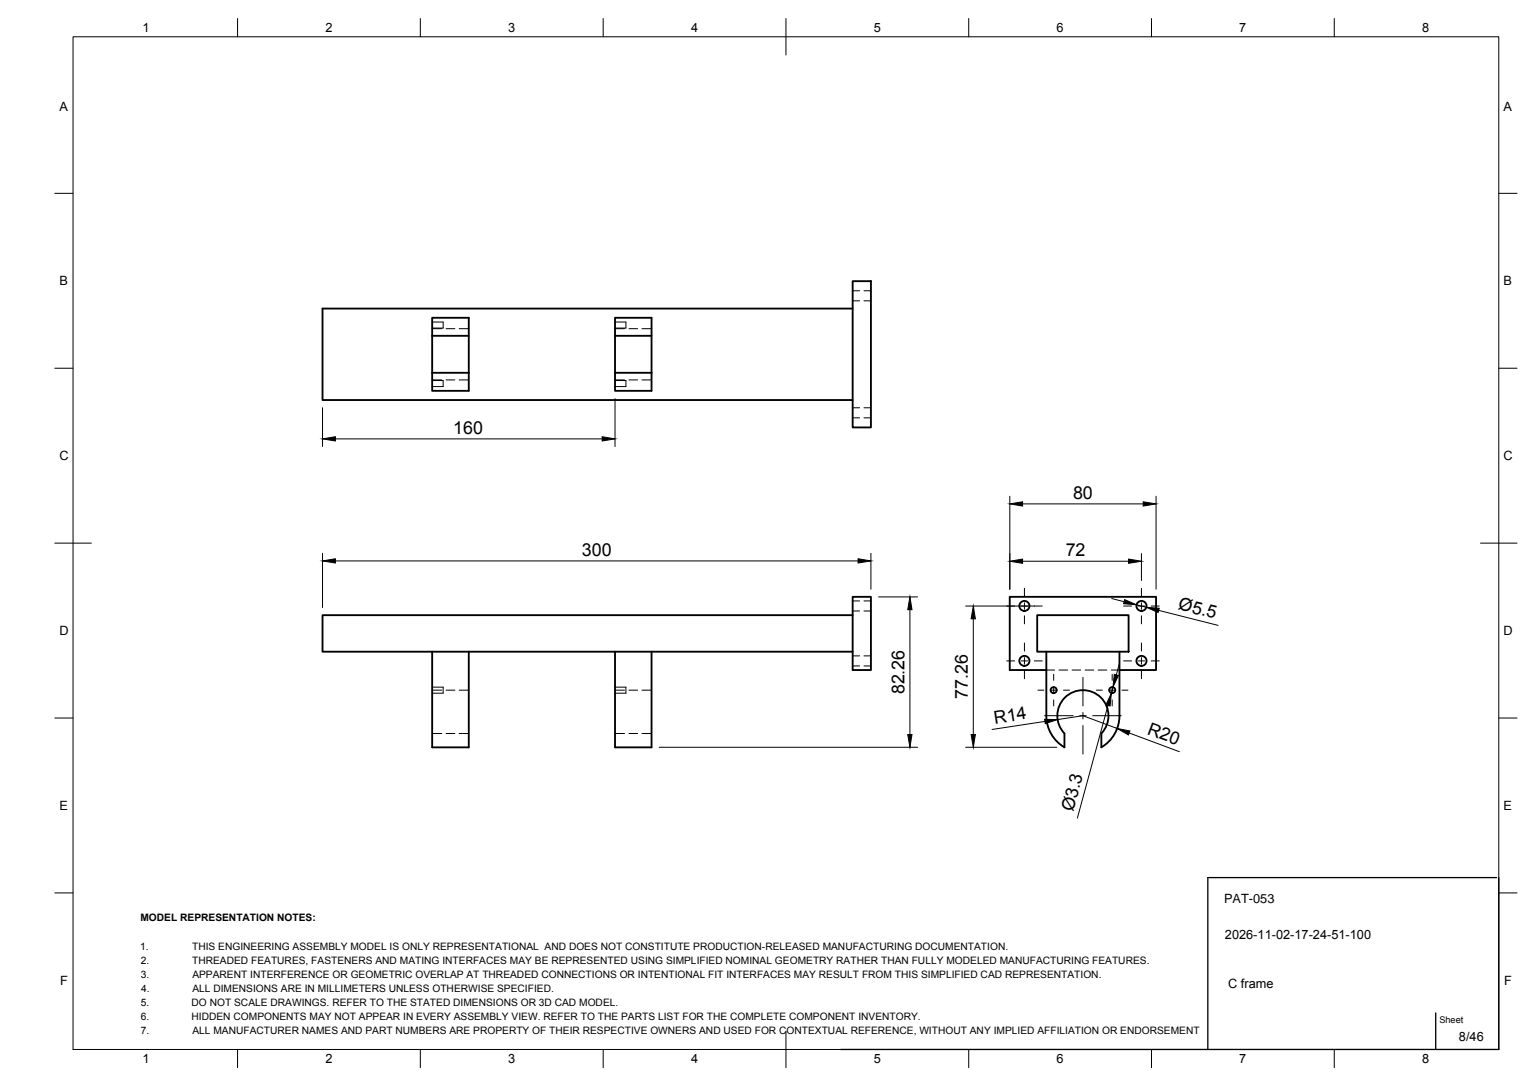
ISO-10303-21;
HEADER;
/* Generated by software containing ST-Developer
 * from STEP Tools, Inc. (www.steptools.com) 
 */

FILE_DESCRIPTION(
/* description */ ('Hand-operated arbor press'),
/* implementation_level */ '2;1');

FILE_NAME(
/* name */ 'C frame.step',
/* time_stamp */ '2026-10-28T03:25:25-07:00',
/* author */ (''),
/* organization */ (''),
/* preprocessor_version */ 'ST-DEVELOPER v20.2',
/* originating_system */ 'Autodesk Translation Framework v15.17.0.0',
/* authorisation */ '');

FILE_SCHEMA (('AUTOMOTIVE_DESIGN { 1 0 10303 214 3 1 1 }'));
ENDSEC;

DATA;
#10=MECHANICAL_DESIGN_GEOMETRIC_PRESENTATION_REPRESENTATION('',(#589),#32751);
#505=SHAPE_REPRESENTATION_RELATIONSHIP('SRR','None',#32934,#547);
#547=ADVANCED_BREP_SHAPE_REPRESENTATION('',(#638),#32708);
#589=STYLED_ITEM('',(#33221),#638);
#638=MANIFOLD_SOLID_BREP('Body1',#12486);
#700=FACE_BOUND('',#2033,.T.);
#701=FACE_BOUND('',#2034,.T.);
#702=FACE_BOUND('',#2048,.T.);
#703=FACE_BOUND('',#2049,.T.);
#704=FACE_BOUND('',#2057,.T.);
#705=FACE_BOUND('',#2058,.T.);
#706=FACE_BOUND('',#2059,.T.);
#707=FACE_BOUND('',#2060,.T.);
#708=FACE_BOUND('',#2061,.T.);
#709=FACE_BOUND('',#2070,.T.);
#710=FACE_BOUND('',#2071,.T.);
#711=FACE_BOUND('',#2074,.T.);
#712=FACE_BOUND('',#2075,.T.);
#713=FACE_BOUND('',#2076,.T.);
#714=FACE_BOUND('',#2077,.T.);
#867=PLANE('',#13056);
#868=PLANE('',#13060);
#869=PLANE('',#13061);
#870=PLANE('',#13062);
#871=PLANE('',#13063);
#872=PLANE('',#13073);
#873=PLANE('',#13074);
#874=PLANE('',#13075);
#875=PLANE('',#13079);
#876=PLANE('',#13083);
#877=PLANE('',#13084);
#878=PLANE('',#13085);
#879=PLANE('',#13086);
#880=PLANE('',#13096);
#881=PLANE('',#13097);
#882=PLANE('',#13098);
#883=PLANE('',#13111);
#884=PLANE('',#13112);
#885=PLANE('',#13113);
#886=PLANE('',#13114);
#887=PLANE('',#13115);
#888=PLANE('',#13116);
#889=PLANE('',#13117);
#890=PLANE('',#13118);
#891=PLANE('',#13119);
#892=PLANE('',#13120);
#893=PLANE('',#13121);
#1321=FACE_OUTER_BOUND('',#2022,.T.);
#1322=FACE_OUTER_BOUND('',#2023,.T.);
#1323=FACE_OUTER_BOUND('',#2024,.T.);
#1324=FACE_OUTER_BOUND('',#2025,.T.);
#1325=FACE_OUTER_BOUND('',#2026,.T.);
#1326=FACE_OUTER_BOUND('',#2027,.T.);
#1327=FACE_OUTER_BOUND('',#2028,.T.);
#1328=FACE_OUTER_BOUND('',#2029,.T.);
#1329=FACE_OUTER_BOUND('',#2030,.T.);
#1330=FACE_OUTER_BOUND('',#2031,.T.);
#1331=FACE_OUTER_BOUND('',#2032,.T.);
#1332=FACE_OUTER_BOUND('',#2035,.T.);
#1333=FACE_OUTER_BOUND('',#2036,.T.);
#1334=FACE_OUTER_BOUND('',#2037,.T.);
#1335=FACE_OUTER_BOUND('',#2038,.T.);
#1336=FACE_OUTER_BOUND('',#2039,.T.);
#1337=FACE_OUTER_BOUND('',#2040,.T.);
#1338=FACE_OUTER_BOUND('',#2041,.T.);
#1339=FACE_OUTER_BOUND('',#2042,.T.);
#1340=FACE_OUTER_BOUND('',#2043,.T.);
#1341=FACE_OUTER_BOUND('',#2044,.T.);
#1342=FACE_OUTER_BOUND('',#2045,.T.);
#1343=FACE_OUTER_BOUND('',#2046,.T.);
#1344=FACE_OUTER_BOUND('',#2047,.T.);
#1345=FACE_OUTER_BOUND('',#2050,.T.);
#1346=FACE_OUTER_BOUND('',#2051,.T.);
#1347=FACE_OUTER_BOUND('',#2052,.T.);
#1348=FACE_OUTER_BOUND('',#2053,.T.);
#1349=FACE_OUTER_BOUND('',#2054,.T.);
#1350=FACE_OUTER_BOUND('',#2055,.T.);
#1351=FACE_OUTER_BOUND('',#2056,.T.);
#1352=FACE_OUTER_BOUND('',#2062,.T.);
#1353=FACE_OUTER_BOUND('',#2063,.T.);
#1354=FACE_OUTER_BOUND('',#2064,.T.);
#1355=FACE_OUTER_BOUND('',#2065,.T.);
#1356=FACE_OUTER_BOUND('',#2066,.T.);
#1357=FACE_OUTER_BOUND('',#2067,.T.);
#1358=FACE_OUTER_BOUND('',#2068,.T.);
#1359=FACE_OUTER_BOUND('',#2069,.T.);
#1360=FACE_OUTER_BOUND('',#2072,.T.);
#1361=FACE_OUTER_BOUND('',#2073,.T.);
#2022=EDGE_LOOP('',(#8456,#8457,#8458,#8459));
#2023=EDGE_LOOP('',(#8460));
#2024=EDGE_LOOP('',(#8461,#8462,#8463,#8464));
#2025=EDGE_LOOP('',(#8465));
#2026=EDGE_LOOP('',(#8466,#8467,#8468,#8469));
#2027=EDGE_LOOP('',(#8470,#8471,#8472,#8473));
#2028=EDGE_LOOP('',(#8474,#8475,#8476,#8477,#8478,#8479,#8480,#8481));
#2029=EDGE_LOOP('',(#8482,#8483,#8484,#8485));
#2030=EDGE_LOOP('',(#8486,#8487,#8488,#8489));
#2031=EDGE_LOOP('',(#8490,#8491,#8492,#8493));
#2032=EDGE_LOOP('',(#8494,#8495,#8496,#8497,#8498,#8499,#8500,#8501));
#2033=EDGE_LOOP('',(#8502));
#2034=EDGE_LOOP('',(#8503));
#2035=EDGE_LOOP('',(#8504,#8505,#8506,#8507));
#2036=EDGE_LOOP('',(#8508,#8509,#8510,#8511));
#2037=EDGE_LOOP('',(#8512,#8513,#8514,#8515));
#2038=EDGE_LOOP('',(#8516));
#2039=EDGE_LOOP('',(#8517,#8518,#8519,#8520));
#2040=EDGE_LOOP('',(#8521));
#2041=EDGE_LOOP('',(#8522,#8523,#8524,#8525));
#2042=EDGE_LOOP('',(#8526,#8527,#8528,#8529));
#2043=EDGE_LOOP('',(#8530,#8531,#8532,#8533,#8534,#8535,#8536,#8537));
#2044=EDGE_LOOP('',(#8538,#8539,#8540,#8541));
#2045=EDGE_LOOP('',(#8542,#8543,#8544,#8545));
#2046=EDGE_LOOP('',(#8546,#8547,#8548,#8549));
#2047=EDGE_LOOP('',(#8550,#8551,#8552,#8553,#8554,#8555,#8556,#8557));
#2048=EDGE_LOOP('',(#8558));
#2049=EDGE_LOOP('',(#8559));
#2050=EDGE_LOOP('',(#8560,#8561,#8562,#8563));
#2051=EDGE_LOOP('',(#8564,#8565,#8566,#8567));
#2052=EDGE_LOOP('',(#8568,#8569,#8570,#8571));
#2053=EDGE_LOOP('',(#8572,#8573,#8574,#8575));
#2054=EDGE_LOOP('',(#8576,#8577,#8578,#8579));
#2055=EDGE_LOOP('',(#8580,#8581,#8582,#8583));
#2056=EDGE_LOOP('',(#8584,#8585,#8586,#8587));
#2057=EDGE_LOOP('',(#8588,#8589,#8590,#8591));
#2058=EDGE_LOOP('',(#8592));
#2059=EDGE_LOOP('',(#8593));
#2060=EDGE_LOOP('',(#8594));
#2061=EDGE_LOOP('',(#8595));
#2062=EDGE_LOOP('',(#8596,#8597,#8598,#8599));
#2063=EDGE_LOOP('',(#8600,#8601,#8602,#8603));
#2064=EDGE_LOOP('',(#8604,#8605,#8606,#8607));
#2065=EDGE_LOOP('',(#8608,#8609,#8610,#8611));
#2066=EDGE_LOOP('',(#8612,#8613,#8614,#8615));
#2067=EDGE_LOOP('',(#8616,#8617,#8618,#8619));
#2068=EDGE_LOOP('',(#8620,#8621,#8622,#8623));
#2069=EDGE_LOOP('',(#8624,#8625,#8626,#8627));
#2070=EDGE_LOOP('',(#8628,#8629,#8630,#8631));
#2071=EDGE_LOOP('',(#8632,#8633,#8634,#8635));
#2072=EDGE_LOOP('',(#8636,#8637,#8638,#8639));
#2073=EDGE_LOOP('',(#8640,#8641,#8642,#8643));
#2074=EDGE_LOOP('',(#8644));
#2075=EDGE_LOOP('',(#8645));
#2076=EDGE_LOOP('',(#8646));
#2077=EDGE_LOOP('',(#8647));
#2870=LINE('',#17786,#4041);
#2871=LINE('',#17793,#4042);
#2872=LINE('',#17799,#4043);
#2873=LINE('',#17801,#4044);
#2874=LINE('',#17803,#4045);
#2875=LINE('',#17804,#4046);
#2876=LINE('',#17808,#4047);
#2877=LINE('',#17810,#4048);
#2878=LINE('',#17812,#4049);
#2879=LINE('',#17813,#4050);
#2880=LINE('',#17818,#4051);
#2881=LINE('',#17820,#4052);
#2882=LINE('',#17822,#4053);
#2883=LINE('',#17829,#4054);
#2884=LINE('',#17834,#4055);
#2885=LINE('',#17837,#4056);
#2886=LINE('',#17839,#4057);
#2887=LINE('',#17840,#4058);
#2888=LINE('',#17842,#4059);
#2889=LINE('',#17844,#4060);
#2890=LINE('',#17849,#4061);
#2891=LINE('',#17856,#4062);
#2892=LINE('',#17862,#4063);
#2893=LINE('',#17864,#4064);
#2894=LINE('',#17866,#4065);
#2895=LINE('',#17867,#4066);
#2896=LINE('',#17871,#4067);
#2897=LINE('',#17873,#4068);
#2898=LINE('',#17875,#4069);
#2899=LINE('',#17876,#4070);
#2900=LINE('',#17881,#4071);
#2901=LINE('',#17883,#4072);
#2902=LINE('',#17885,#4073);
#2903=LINE('',#17892,#4074);
#2904=LINE('',#17897,#4075);
#2905=LINE('',#17900,#4076);
#2906=LINE('',#17902,#4077);
#2907=LINE('',#17903,#4078);
#2908=LINE('',#17905,#4079);
#2909=LINE('',#17907,#4080);
#2910=LINE('',#17912,#4081);
#2911=LINE('',#17918,#4082);
#2912=LINE('',#17924,#4083);
#2913=LINE('',#17930,#4084);
#2914=LINE('',#17935,#4085);
#2915=LINE('',#17937,#4086);
#2916=LINE('',#17939,#4087);
#2917=LINE('',#17940,#4088);
#2918=LINE('',#17943,#4089);
#2919=LINE('',#17945,#4090);
#2920=LINE('',#17947,#4091);
#2921=LINE('',#17948,#4092);
#2922=LINE('',#17952,#4093);
#2923=LINE('',#17953,#4094);
#2924=LINE('',#17954,#4095);
#2925=LINE('',#17957,#4096);
#2926=LINE('',#17958,#4097);
#2927=LINE('',#17961,#4098);
#2928=LINE('',#17962,#4099);
#2929=LINE('',#17964,#4100);
#2930=LINE('',#17967,#4101);
#2931=LINE('',#17969,#4102);
#2932=LINE('',#17970,#4103);
#2933=LINE('',#17973,#4104);
#2934=LINE('',#17974,#4105);
#2935=LINE('',#17977,#4106);
#2936=LINE('',#17978,#4107);
#2937=LINE('',#17980,#4108);
#4041=VECTOR('',#14313,0.165);
#4042=VECTOR('',#14322,0.165);
#4043=VECTOR('',#14329,1.);
#4044=VECTOR('',#14330,1.);
#4045=VECTOR('',#14331,1.);
#4046=VECTOR('',#14332,1.);
#4047=VECTOR('',#14335,1.);
#4048=VECTOR('',#14336,1.);
#4049=VECTOR('',#14337,1.);
#4050=VECTOR('',#14338,1.);
#4051=VECTOR('',#14343,1.);
#4052=VECTOR('',#14344,1.);
#4053=VECTOR('',#14345,1.);
#4054=VECTOR('',#14356,1.);
#4055=VECTOR('',#14363,1.);
#4056=VECTOR('',#14366,1.);
#4057=VECTOR('',#14367,1.);
#4058=VECTOR('',#14368,1.);
#4059=VECTOR('',#14371,1.);
#4060=VECTOR('',#14374,1.);
#4061=VECTOR('',#14379,0.165);
#4062=VECTOR('',#14388,0.165);
#4063=VECTOR('',#14395,1.);
#4064=VECTOR('',#14396,1.);
#4065=VECTOR('',#14397,1.);
#4066=VECTOR('',#14398,1.);
#4067=VECTOR('',#14401,1.);
#4068=VECTOR('',#14402,1.);
#4069=VECTOR('',#14403,1.);
#4070=VECTOR('',#14404,1.);
#4071=VECTOR('',#14409,1.);
#4072=VECTOR('',#14410,1.);
#4073=VECTOR('',#14411,1.);
#4074=VECTOR('',#14422,1.);
#4075=VECTOR('',#14429,1.);
#4076=VECTOR('',#14432,1.);
#4077=VECTOR('',#14433,1.);
#4078=VECTOR('',#14434,1.);
#4079=VECTOR('',#14437,1.);
#4080=VECTOR('',#14440,1.);
#4081=VECTOR('',#14445,0.275);
#4082=VECTOR('',#14452,0.275);
#4083=VECTOR('',#14459,0.275);
#4084=VECTOR('',#14466,0.275);
#4085=VECTOR('',#14471,1.);
#4086=VECTOR('',#14472,1.);
#4087=VECTOR('',#14473,1.);
#4088=VECTOR('',#14474,1.);
#4089=VECTOR('',#14475,1.);
#4090=VECTOR('',#14476,1.);
#4091=VECTOR('',#14477,1.);
#4092=VECTOR('',#14478,1.);
#4093=VECTOR('',#14481,1.);
#4094=VECTOR('',#14482,1.);
#4095=VECTOR('',#14483,1.);
#4096=VECTOR('',#14486,1.);
#4097=VECTOR('',#14487,1.);
#4098=VECTOR('',#14490,1.);
#4099=VECTOR('',#14491,1.);
#4100=VECTOR('',#14494,1.);
#4101=VECTOR('',#14497,1.);
#4102=VECTOR('',#14498,1.);
#4103=VECTOR('',#14499,1.);
#4104=VECTOR('',#14502,1.);
#4105=VECTOR('',#14503,1.);
#4106=VECTOR('',#14506,1.);
#4107=VECTOR('',#14507,1.);
#4108=VECTOR('',#14510,1.);
#5186=CIRCLE('',#13054,0.165);
#5187=CIRCLE('',#13055,0.165);
#5188=CIRCLE('',#13058,0.165);
#5189=CIRCLE('',#13059,0.165);
#5190=CIRCLE('',#13064,2.);
#5191=CIRCLE('',#13065,2.);
#5192=CIRCLE('',#13066,1.4);
#5193=CIRCLE('',#13068,1.4);
#5194=CIRCLE('',#13070,2.);
#5195=CIRCLE('',#13072,2.);
#5196=CIRCLE('',#13077,0.165);
#5197=CIRCLE('',#13078,0.165);
#5198=CIRCLE('',#13081,0.165);
#5199=CIRCLE('',#13082,0.165);
#5200=CIRCLE('',#13087,2.);
#5201=CIRCLE('',#13088,2.);
#5202=CIRCLE('',#13089,1.4);
#5203=CIRCLE('',#13091,1.4);
#5204=CIRCLE('',#13093,2.);
#5205=CIRCLE('',#13095,2.);
#5206=CIRCLE('',#13100,0.275);
#5207=CIRCLE('',#13101,0.275);
#5208=CIRCLE('',#13103,0.275);
#5209=CIRCLE('',#13104,0.275);
#5210=CIRCLE('',#13106,0.275);
#5211=CIRCLE('',#13107,0.275);
#5212=CIRCLE('',#13109,0.275);
#5213=CIRCLE('',#13110,0.275);
#5600=VERTEX_POINT('',#17783);
#5601=VERTEX_POINT('',#17785);
#5602=VERTEX_POINT('',#17790);
#5603=VERTEX_POINT('',#17792);
#5604=VERTEX_POINT('',#17797);
#5605=VERTEX_POINT('',#17798);
#5606=VERTEX_POINT('',#17800);
#5607=VERTEX_POINT('',#17802);
#5608=VERTEX_POINT('',#17806);
#5609=VERTEX_POINT('',#17807);
#5610=VERTEX_POINT('',#17809);
#5611=VERTEX_POINT('',#17811);
#5612=VERTEX_POINT('',#17815);
#5613=VERTEX_POINT('',#17817);
#5614=VERTEX_POINT('',#17819);
#5615=VERTEX_POINT('',#17821);
#5616=VERTEX_POINT('',#17828);
#5617=VERTEX_POINT('',#17832);
#5618=VERTEX_POINT('',#17836);
#5619=VERTEX_POINT('',#17838);
#5620=VERTEX_POINT('',#17846);
#5621=VERTEX_POINT('',#17848);
#5622=VERTEX_POINT('',#17853);
#5623=VERTEX_POINT('',#17855);
#5624=VERTEX_POINT('',#17860);
#5625=VERTEX_POINT('',#17861);
#5626=VERTEX_POINT('',#17863);
#5627=VERTEX_POINT('',#17865);
#5628=VERTEX_POINT('',#17869);
#5629=VERTEX_POINT('',#17870);
#5630=VERTEX_POINT('',#17872);
#5631=VERTEX_POINT('',#17874);
#5632=VERTEX_POINT('',#17878);
#5633=VERTEX_POINT('',#17880);
#5634=VERTEX_POINT('',#17882);
#5635=VERTEX_POINT('',#17884);
#5636=VERTEX_POINT('',#17891);
#5637=VERTEX_POINT('',#17895);
#5638=VERTEX_POINT('',#17899);
#5639=VERTEX_POINT('',#17901);
#5640=VERTEX_POINT('',#17909);
#5641=VERTEX_POINT('',#17911);
#5642=VERTEX_POINT('',#17915);
#5643=VERTEX_POINT('',#17917);
#5644=VERTEX_POINT('',#17921);
#5645=VERTEX_POINT('',#17923);
#5646=VERTEX_POINT('',#17927);
#5647=VERTEX_POINT('',#17929);
#5648=VERTEX_POINT('',#17933);
#5649=VERTEX_POINT('',#17934);
#5650=VERTEX_POINT('',#17936);
#5651=VERTEX_POINT('',#17938);
#5652=VERTEX_POINT('',#17941);
#5653=VERTEX_POINT('',#17942);
#5654=VERTEX_POINT('',#17944);
#5655=VERTEX_POINT('',#17946);
#5656=VERTEX_POINT('',#17950);
#5657=VERTEX_POINT('',#17951);
#5658=VERTEX_POINT('',#17956);
#5659=VERTEX_POINT('',#17960);
#5660=VERTEX_POINT('',#17966);
#5661=VERTEX_POINT('',#17968);
#5662=VERTEX_POINT('',#17972);
#5663=VERTEX_POINT('',#17976);
#6731=EDGE_CURVE('',#5600,#5600,#5186,.T.);
#6732=EDGE_CURVE('',#5600,#5601,#2870,.T.);
#6733=EDGE_CURVE('',#5601,#5601,#5187,.T.);
#6734=EDGE_CURVE('',#5602,#5602,#5188,.T.);
#6735=EDGE_CURVE('',#5602,#5603,#2871,.T.);
#6736=EDGE_CURVE('',#5603,#5603,#5189,.T.);
#6737=EDGE_CURVE('',#5604,#5605,#2872,.T.);
#6738=EDGE_CURVE('',#5606,#5604,#2873,.T.);
#6739=EDGE_CURVE('',#5607,#5606,#2874,.T.);
#6740=EDGE_CURVE('',#5605,#5607,#2875,.T.);
#6741=EDGE_CURVE('',#5608,#5609,#2876,.T.);
#6742=EDGE_CURVE('',#5610,#5608,#2877,.T.);
#6743=EDGE_CURVE('',#5611,#5610,#2878,.T.);
#6744=EDGE_CURVE('',#5609,#5611,#2879,.T.);
#6745=EDGE_CURVE('',#5612,#5604,#5190,.T.);
#6746=EDGE_CURVE('',#5613,#5612,#2880,.T.);
#6747=EDGE_CURVE('',#5614,#5613,#2881,.T.);
#6748=EDGE_CURVE('',#5615,#5614,#2882,.T.);
#6749=EDGE_CURVE('',#5609,#5615,#5191,.T.);
#6750=EDGE_CURVE('',#5611,#5606,#5192,.T.);
#6751=EDGE_CURVE('',#5607,#5610,#5193,.T.);
#6752=EDGE_CURVE('',#5615,#5616,#2883,.T.);
#6753=EDGE_CURVE('',#5608,#5616,#5194,.T.);
#6754=EDGE_CURVE('',#5617,#5605,#5195,.T.);
#6755=EDGE_CURVE('',#5612,#5617,#2884,.T.);
#6756=EDGE_CURVE('',#5616,#5618,#2885,.T.);
#6757=EDGE_CURVE('',#5619,#5618,#2886,.T.);
#6758=EDGE_CURVE('',#5619,#5617,#2887,.T.);
#6759=EDGE_CURVE('',#5618,#5614,#2888,.T.);
#6760=EDGE_CURVE('',#5613,#5619,#2889,.T.);
#6761=EDGE_CURVE('',#5620,#5620,#5196,.T.);
#6762=EDGE_CURVE('',#5620,#5621,#2890,.T.);
#6763=EDGE_CURVE('',#5621,#5621,#5197,.T.);
#6764=EDGE_CURVE('',#5622,#5622,#5198,.T.);
#6765=EDGE_CURVE('',#5622,#5623,#2891,.T.);
#6766=EDGE_CURVE('',#5623,#5623,#5199,.T.);
#6767=EDGE_CURVE('',#5624,#5625,#2892,.T.);
#6768=EDGE_CURVE('',#5626,#5624,#2893,.T.);
#6769=EDGE_CURVE('',#5627,#5626,#2894,.T.);
#6770=EDGE_CURVE('',#5625,#5627,#2895,.T.);
#6771=EDGE_CURVE('',#5628,#5629,#2896,.T.);
#6772=EDGE_CURVE('',#5630,#5628,#2897,.T.);
#6773=EDGE_CURVE('',#5631,#5630,#2898,.T.);
#6774=EDGE_CURVE('',#5629,#5631,#2899,.T.);
#6775=EDGE_CURVE('',#5632,#5624,#5200,.T.);
#6776=EDGE_CURVE('',#5633,#5632,#2900,.T.);
#6777=EDGE_CURVE('',#5634,#5633,#2901,.T.);
#6778=EDGE_CURVE('',#5635,#5634,#2902,.T.);
#6779=EDGE_CURVE('',#5629,#5635,#5201,.T.);
#6780=EDGE_CURVE('',#5631,#5626,#5202,.T.);
#6781=EDGE_CURVE('',#5627,#5630,#5203,.T.);
#6782=EDGE_CURVE('',#5635,#5636,#2903,.T.);
#6783=EDGE_CURVE('',#5628,#5636,#5204,.T.);
#6784=EDGE_CURVE('',#5637,#5625,#5205,.T.);
#6785=EDGE_CURVE('',#5632,#5637,#2904,.T.);
#6786=EDGE_CURVE('',#5636,#5638,#2905,.T.);
#6787=EDGE_CURVE('',#5639,#5638,#2906,.T.);
#6788=EDGE_CURVE('',#5639,#5637,#2907,.T.);
#6789=EDGE_CURVE('',#5638,#5634,#2908,.T.);
#6790=EDGE_CURVE('',#5633,#5639,#2909,.T.);
#6791=EDGE_CURVE('',#5640,#5640,#5206,.T.);
#6792=EDGE_CURVE('',#5640,#5641,#2910,.T.);
#6793=EDGE_CURVE('',#5641,#5641,#5207,.T.);
#6794=EDGE_CURVE('',#5642,#5642,#5208,.T.);
#6795=EDGE_CURVE('',#5642,#5643,#2911,.T.);
#6796=EDGE_CURVE('',#5643,#5643,#5209,.T.);
#6797=EDGE_CURVE('',#5644,#5644,#5210,.T.);
#6798=EDGE_CURVE('',#5644,#5645,#2912,.T.);
#6799=EDGE_CURVE('',#5645,#5645,#5211,.T.);
#6800=EDGE_CURVE('',#5646,#5646,#5212,.T.);
#6801=EDGE_CURVE('',#5646,#5647,#2913,.T.);
#6802=EDGE_CURVE('',#5647,#5647,#5213,.T.);
#6803=EDGE_CURVE('',#5648,#5649,#2914,.T.);
#6804=EDGE_CURVE('',#5649,#5650,#2915,.T.);
#6805=EDGE_CURVE('',#5650,#5651,#2916,.T.);
#6806=EDGE_CURVE('',#5651,#5648,#2917,.T.);
#6807=EDGE_CURVE('',#5652,#5653,#2918,.T.);
#6808=EDGE_CURVE('',#5654,#5652,#2919,.T.);
#6809=EDGE_CURVE('',#5655,#5654,#2920,.T.);
#6810=EDGE_CURVE('',#5653,#5655,#2921,.T.);
#6811=EDGE_CURVE('',#5656,#5657,#2922,.T.);
#6812=EDGE_CURVE('',#5657,#5648,#2923,.T.);
#6813=EDGE_CURVE('',#5656,#5651,#2924,.T.);
#6814=EDGE_CURVE('',#5658,#5656,#2925,.T.);
#6815=EDGE_CURVE('',#5658,#5650,#2926,.T.);
#6816=EDGE_CURVE('',#5659,#5658,#2927,.T.);
#6817=EDGE_CURVE('',#5659,#5649,#2928,.T.);
#6818=EDGE_CURVE('',#5657,#5659,#2929,.T.);
#6819=EDGE_CURVE('',#5654,#5660,#2930,.T.);
#6820=EDGE_CURVE('',#5661,#5660,#2931,.T.);
#6821=EDGE_CURVE('',#5655,#5661,#2932,.T.);
#6822=EDGE_CURVE('',#5652,#5662,#2933,.T.);
#6823=EDGE_CURVE('',#5660,#5662,#2934,.T.);
#6824=EDGE_CURVE('',#5653,#5663,#2935,.T.);
#6825=EDGE_CURVE('',#5662,#5663,#2936,.T.);
#6826=EDGE_CURVE('',#5663,#5661,#2937,.T.);
#8456=ORIENTED_EDGE('',*,*,#6731,.F.);
#8457=ORIENTED_EDGE('',*,*,#6732,.T.);
#8458=ORIENTED_EDGE('',*,*,#6733,.F.);
#8459=ORIENTED_EDGE('',*,*,#6732,.F.);
#8460=ORIENTED_EDGE('',*,*,#6731,.T.);
#8461=ORIENTED_EDGE('',*,*,#6734,.F.);
#8462=ORIENTED_EDGE('',*,*,#6735,.T.);
#8463=ORIENTED_EDGE('',*,*,#6736,.F.);
#8464=ORIENTED_EDGE('',*,*,#6735,.F.);
#8465=ORIENTED_EDGE('',*,*,#6734,.T.);
#8466=ORIENTED_EDGE('',*,*,#6737,.F.);
#8467=ORIENTED_EDGE('',*,*,#6738,.F.);
#8468=ORIENTED_EDGE('',*,*,#6739,.F.);
#8469=ORIENTED_EDGE('',*,*,#6740,.F.);
#8470=ORIENTED_EDGE('',*,*,#6741,.F.);
#8471=ORIENTED_EDGE('',*,*,#6742,.F.);
#8472=ORIENTED_EDGE('',*,*,#6743,.F.);
#8473=ORIENTED_EDGE('',*,*,#6744,.F.);
#8474=ORIENTED_EDGE('',*,*,#6738,.T.);
#8475=ORIENTED_EDGE('',*,*,#6745,.F.);
#8476=ORIENTED_EDGE('',*,*,#6746,.F.);
#8477=ORIENTED_EDGE('',*,*,#6747,.F.);
#8478=ORIENTED_EDGE('',*,*,#6748,.F.);
#8479=ORIENTED_EDGE('',*,*,#6749,.F.);
#8480=ORIENTED_EDGE('',*,*,#6744,.T.);
#8481=ORIENTED_EDGE('',*,*,#6750,.T.);
#8482=ORIENTED_EDGE('',*,*,#6739,.T.);
#8483=ORIENTED_EDGE('',*,*,#6750,.F.);
#8484=ORIENTED_EDGE('',*,*,#6743,.T.);
#8485=ORIENTED_EDGE('',*,*,#6751,.F.);
#8486=ORIENTED_EDGE('',*,*,#6741,.T.);
#8487=ORIENTED_EDGE('',*,*,#6749,.T.);
#8488=ORIENTED_EDGE('',*,*,#6752,.T.);
#8489=ORIENTED_EDGE('',*,*,#6753,.F.);
#8490=ORIENTED_EDGE('',*,*,#6737,.T.);
#8491=ORIENTED_EDGE('',*,*,#6754,.F.);
#8492=ORIENTED_EDGE('',*,*,#6755,.F.);
#8493=ORIENTED_EDGE('',*,*,#6745,.T.);
#8494=ORIENTED_EDGE('',*,*,#6740,.T.);
#8495=ORIENTED_EDGE('',*,*,#6751,.T.);
#8496=ORIENTED_EDGE('',*,*,#6742,.T.);
#8497=ORIENTED_EDGE('',*,*,#6753,.T.);
#8498=ORIENTED_EDGE('',*,*,#6756,.T.);
#8499=ORIENTED_EDGE('',*,*,#6757,.F.);
#8500=ORIENTED_EDGE('',*,*,#6758,.T.);
#8501=ORIENTED_EDGE('',*,*,#6754,.T.);
#8502=ORIENTED_EDGE('',*,*,#6733,.T.);
#8503=ORIENTED_EDGE('',*,*,#6736,.T.);
#8504=ORIENTED_EDGE('',*,*,#6759,.F.);
#8505=ORIENTED_EDGE('',*,*,#6756,.F.);
#8506=ORIENTED_EDGE('',*,*,#6752,.F.);
#8507=ORIENTED_EDGE('',*,*,#6748,.T.);
#8508=ORIENTED_EDGE('',*,*,#6760,.F.);
#8509=ORIENTED_EDGE('',*,*,#6746,.T.);
#8510=ORIENTED_EDGE('',*,*,#6755,.T.);
#8511=ORIENTED_EDGE('',*,*,#6758,.F.);
#8512=ORIENTED_EDGE('',*,*,#6761,.F.);
#8513=ORIENTED_EDGE('',*,*,#6762,.T.);
#8514=ORIENTED_EDGE('',*,*,#6763,.F.);
#8515=ORIENTED_EDGE('',*,*,#6762,.F.);
#8516=ORIENTED_EDGE('',*,*,#6761,.T.);
#8517=ORIENTED_EDGE('',*,*,#6764,.F.);
#8518=ORIENTED_EDGE('',*,*,#6765,.T.);
#8519=ORIENTED_EDGE('',*,*,#6766,.F.);
#8520=ORIENTED_EDGE('',*,*,#6765,.F.);
#8521=ORIENTED_EDGE('',*,*,#6764,.T.);
#8522=ORIENTED_EDGE('',*,*,#6767,.F.);
#8523=ORIENTED_EDGE('',*,*,#6768,.F.);
#8524=ORIENTED_EDGE('',*,*,#6769,.F.);
#8525=ORIENTED_EDGE('',*,*,#6770,.F.);
#8526=ORIENTED_EDGE('',*,*,#6771,.F.);
#8527=ORIENTED_EDGE('',*,*,#6772,.F.);
#8528=ORIENTED_EDGE('',*,*,#6773,.F.);
#8529=ORIENTED_EDGE('',*,*,#6774,.F.);
#8530=ORIENTED_EDGE('',*,*,#6768,.T.);
#8531=ORIENTED_EDGE('',*,*,#6775,.F.);
#8532=ORIENTED_EDGE('',*,*,#6776,.F.);
#8533=ORIENTED_EDGE('',*,*,#6777,.F.);
#8534=ORIENTED_EDGE('',*,*,#6778,.F.);
#8535=ORIENTED_EDGE('',*,*,#6779,.F.);
#8536=ORIENTED_EDGE('',*,*,#6774,.T.);
#8537=ORIENTED_EDGE('',*,*,#6780,.T.);
#8538=ORIENTED_EDGE('',*,*,#6769,.T.);
#8539=ORIENTED_EDGE('',*,*,#6780,.F.);
#8540=ORIENTED_EDGE('',*,*,#6773,.T.);
#8541=ORIENTED_EDGE('',*,*,#6781,.F.);
#8542=ORIENTED_EDGE('',*,*,#6771,.T.);
#8543=ORIENTED_EDGE('',*,*,#6779,.T.);
#8544=ORIENTED_EDGE('',*,*,#6782,.T.);
#8545=ORIENTED_EDGE('',*,*,#6783,.F.);
#8546=ORIENTED_EDGE('',*,*,#6767,.T.);
#8547=ORIENTED_EDGE('',*,*,#6784,.F.);
#8548=ORIENTED_EDGE('',*,*,#6785,.F.);
#8549=ORIENTED_EDGE('',*,*,#6775,.T.);
#8550=ORIENTED_EDGE('',*,*,#6770,.T.);
#8551=ORIENTED_EDGE('',*,*,#6781,.T.);
#8552=ORIENTED_EDGE('',*,*,#6772,.T.);
#8553=ORIENTED_EDGE('',*,*,#6783,.T.);
#8554=ORIENTED_EDGE('',*,*,#6786,.T.);
#8555=ORIENTED_EDGE('',*,*,#6787,.F.);
#8556=ORIENTED_EDGE('',*,*,#6788,.T.);
#8557=ORIENTED_EDGE('',*,*,#6784,.T.);
#8558=ORIENTED_EDGE('',*,*,#6763,.T.);
#8559=ORIENTED_EDGE('',*,*,#6766,.T.);
#8560=ORIENTED_EDGE('',*,*,#6789,.F.);
#8561=ORIENTED_EDGE('',*,*,#6786,.F.);
#8562=ORIENTED_EDGE('',*,*,#6782,.F.);
#8563=ORIENTED_EDGE('',*,*,#6778,.T.);
#8564=ORIENTED_EDGE('',*,*,#6790,.F.);
#8565=ORIENTED_EDGE('',*,*,#6776,.T.);
#8566=ORIENTED_EDGE('',*,*,#6785,.T.);
#8567=ORIENTED_EDGE('',*,*,#6788,.F.);
#8568=ORIENTED_EDGE('',*,*,#6791,.F.);
#8569=ORIENTED_EDGE('',*,*,#6792,.T.);
#8570=ORIENTED_EDGE('',*,*,#6793,.F.);
#8571=ORIENTED_EDGE('',*,*,#6792,.F.);
#8572=ORIENTED_EDGE('',*,*,#6794,.F.);
#8573=ORIENTED_EDGE('',*,*,#6795,.T.);
#8574=ORIENTED_EDGE('',*,*,#6796,.F.);
#8575=ORIENTED_EDGE('',*,*,#6795,.F.);
#8576=ORIENTED_EDGE('',*,*,#6797,.F.);
#8577=ORIENTED_EDGE('',*,*,#6798,.T.);
#8578=ORIENTED_EDGE('',*,*,#6799,.F.);
#8579=ORIENTED_EDGE('',*,*,#6798,.F.);
#8580=ORIENTED_EDGE('',*,*,#6800,.F.);
#8581=ORIENTED_EDGE('',*,*,#6801,.T.);
#8582=ORIENTED_EDGE('',*,*,#6802,.F.);
#8583=ORIENTED_EDGE('',*,*,#6801,.F.);
#8584=ORIENTED_EDGE('',*,*,#6803,.T.);
#8585=ORIENTED_EDGE('',*,*,#6804,.T.);
#8586=ORIENTED_EDGE('',*,*,#6805,.T.);
#8587=ORIENTED_EDGE('',*,*,#6806,.T.);
#8588=ORIENTED_EDGE('',*,*,#6807,.F.);
#8589=ORIENTED_EDGE('',*,*,#6808,.F.);
#8590=ORIENTED_EDGE('',*,*,#6809,.F.);
#8591=ORIENTED_EDGE('',*,*,#6810,.F.);
#8592=ORIENTED_EDGE('',*,*,#6802,.T.);
#8593=ORIENTED_EDGE('',*,*,#6799,.T.);
#8594=ORIENTED_EDGE('',*,*,#6796,.T.);
#8595=ORIENTED_EDGE('',*,*,#6793,.T.);
#8596=ORIENTED_EDGE('',*,*,#6811,.T.);
#8597=ORIENTED_EDGE('',*,*,#6812,.T.);
#8598=ORIENTED_EDGE('',*,*,#6806,.F.);
#8599=ORIENTED_EDGE('',*,*,#6813,.F.);
#8600=ORIENTED_EDGE('',*,*,#6814,.T.);
#8601=ORIENTED_EDGE('',*,*,#6813,.T.);
#8602=ORIENTED_EDGE('',*,*,#6805,.F.);
#8603=ORIENTED_EDGE('',*,*,#6815,.F.);
#8604=ORIENTED_EDGE('',*,*,#6816,.T.);
#8605=ORIENTED_EDGE('',*,*,#6815,.T.);
#8606=ORIENTED_EDGE('',*,*,#6804,.F.);
#8607=ORIENTED_EDGE('',*,*,#6817,.F.);
#8608=ORIENTED_EDGE('',*,*,#6818,.T.);
#8609=ORIENTED_EDGE('',*,*,#6817,.T.);
#8610=ORIENTED_EDGE('',*,*,#6803,.F.);
#8611=ORIENTED_EDGE('',*,*,#6812,.F.);
#8612=ORIENTED_EDGE('',*,*,#6809,.T.);
#8613=ORIENTED_EDGE('',*,*,#6819,.T.);
#8614=ORIENTED_EDGE('',*,*,#6820,.F.);
#8615=ORIENTED_EDGE('',*,*,#6821,.F.);
#8616=ORIENTED_EDGE('',*,*,#6808,.T.);
#8617=ORIENTED_EDGE('',*,*,#6822,.T.);
#8618=ORIENTED_EDGE('',*,*,#6823,.F.);
#8619=ORIENTED_EDGE('',*,*,#6819,.F.);
#8620=ORIENTED_EDGE('',*,*,#6807,.T.);
#8621=ORIENTED_EDGE('',*,*,#6824,.T.);
#8622=ORIENTED_EDGE('',*,*,#6825,.F.);
#8623=ORIENTED_EDGE('',*,*,#6822,.F.);
#8624=ORIENTED_EDGE('',*,*,#6810,.T.);
#8625=ORIENTED_EDGE('',*,*,#6821,.T.);
#8626=ORIENTED_EDGE('',*,*,#6826,.F.);
#8627=ORIENTED_EDGE('',*,*,#6824,.F.);
#8628=ORIENTED_EDGE('',*,*,#6759,.T.);
#8629=ORIENTED_EDGE('',*,*,#6747,.T.);
#8630=ORIENTED_EDGE('',*,*,#6760,.T.);
#8631=ORIENTED_EDGE('',*,*,#6757,.T.);
#8632=ORIENTED_EDGE('',*,*,#6789,.T.);
#8633=ORIENTED_EDGE('',*,*,#6777,.T.);
#8634=ORIENTED_EDGE('',*,*,#6790,.T.);
#8635=ORIENTED_EDGE('',*,*,#6787,.T.);
#8636=ORIENTED_EDGE('',*,*,#6826,.T.);
#8637=ORIENTED_EDGE('',*,*,#6820,.T.);
#8638=ORIENTED_EDGE('',*,*,#6823,.T.);
#8639=ORIENTED_EDGE('',*,*,#6825,.T.);
#8640=ORIENTED_EDGE('',*,*,#6818,.F.);
#8641=ORIENTED_EDGE('',*,*,#6811,.F.);
#8642=ORIENTED_EDGE('',*,*,#6814,.F.);
#8643=ORIENTED_EDGE('',*,*,#6816,.F.);
#8644=ORIENTED_EDGE('',*,*,#6791,.T.);
#8645=ORIENTED_EDGE('',*,*,#6794,.T.);
#8646=ORIENTED_EDGE('',*,*,#6797,.T.);
#8647=ORIENTED_EDGE('',*,*,#6800,.T.);
#11652=CYLINDRICAL_SURFACE('',#13053,0.165);
#11653=CYLINDRICAL_SURFACE('',#13057,0.165);
#11654=CYLINDRICAL_SURFACE('',#13067,1.4);
#11655=CYLINDRICAL_SURFACE('',#13069,2.);
#11656=CYLINDRICAL_SURFACE('',#13071,2.);
#11657=CYLINDRICAL_SURFACE('',#13076,0.165);
#11658=CYLINDRICAL_SURFACE('',#13080,0.165);
#11659=CYLINDRICAL_SURFACE('',#13090,1.4);
#11660=CYLINDRICAL_SURFACE('',#13092,2.);
#11661=CYLINDRICAL_SURFACE('',#13094,2.);
#11662=CYLINDRICAL_SURFACE('',#13099,0.275);
#11663=CYLINDRICAL_SURFACE('',#13102,0.275);
#11664=CYLINDRICAL_SURFACE('',#13105,0.275);
#11665=CYLINDRICAL_SURFACE('',#13108,0.275);
#11830=ADVANCED_FACE('',(#1321),#11652,.F.);
#11831=ADVANCED_FACE('',(#1322),#867,.T.);
#11832=ADVANCED_FACE('',(#1323),#11653,.F.);
#11833=ADVANCED_FACE('',(#1324),#868,.T.);
#11834=ADVANCED_FACE('',(#1325),#869,.F.);
#11835=ADVANCED_FACE('',(#1326),#870,.F.);
#11836=ADVANCED_FACE('',(#1327),#871,.F.);
#11837=ADVANCED_FACE('',(#1328),#11654,.F.);
#11838=ADVANCED_FACE('',(#1329),#11655,.T.);
#11839=ADVANCED_FACE('',(#1330),#11656,.T.);
#11840=ADVANCED_FACE('',(#1331,#700,#701),#872,.T.);
#11841=ADVANCED_FACE('',(#1332),#873,.T.);
#11842=ADVANCED_FACE('',(#1333),#874,.T.);
#11843=ADVANCED_FACE('',(#1334),#11657,.F.);
#11844=ADVANCED_FACE('',(#1335),#875,.T.);
#11845=ADVANCED_FACE('',(#1336),#11658,.F.);
#11846=ADVANCED_FACE('',(#1337),#876,.T.);
#11847=ADVANCED_FACE('',(#1338),#877,.F.);
#11848=ADVANCED_FACE('',(#1339),#878,.F.);
#11849=ADVANCED_FACE('',(#1340),#879,.F.);
#11850=ADVANCED_FACE('',(#1341),#11659,.F.);
#11851=ADVANCED_FACE('',(#1342),#11660,.T.);
#11852=ADVANCED_FACE('',(#1343),#11661,.T.);
#11853=ADVANCED_FACE('',(#1344,#702,#703),#880,.T.);
#11854=ADVANCED_FACE('',(#1345),#881,.T.);
#11855=ADVANCED_FACE('',(#1346),#882,.T.);
#11856=ADVANCED_FACE('',(#1347),#11662,.F.);
#11857=ADVANCED_FACE('',(#1348),#11663,.F.);
#11858=ADVANCED_FACE('',(#1349),#11664,.F.);
#11859=ADVANCED_FACE('',(#1350),#11665,.F.);
#11860=ADVANCED_FACE('',(#1351,#704,#705,#706,#707,#708),#883,.T.);
#11861=ADVANCED_FACE('',(#1352),#884,.T.);
#11862=ADVANCED_FACE('',(#1353),#885,.T.);
#11863=ADVANCED_FACE('',(#1354),#886,.T.);
#11864=ADVANCED_FACE('',(#1355),#887,.T.);
#11865=ADVANCED_FACE('',(#1356),#888,.T.);
#11866=ADVANCED_FACE('',(#1357),#889,.T.);
#11867=ADVANCED_FACE('',(#1358),#890,.T.);
#11868=ADVANCED_FACE('',(#1359,#709,#710),#891,.T.);
#11869=ADVANCED_FACE('',(#1360),#892,.T.);
#11870=ADVANCED_FACE('',(#1361,#711,#712,#713,#714),#893,.F.);
#12486=CLOSED_SHELL('',(#11830,#11831,#11832,#11833,#11834,#11835,#11836,
#11837,#11838,#11839,#11840,#11841,#11842,#11843,#11844,#11845,#11846,#11847,
#11848,#11849,#11850,#11851,#11852,#11853,#11854,#11855,#11856,#11857,#11858,
#11859,#11860,#11861,#11862,#11863,#11864,#11865,#11866,#11867,#11868,#11869,
#11870));
#13052=AXIS2_PLACEMENT_3D('',#17781,#14307,#14308);
#13053=AXIS2_PLACEMENT_3D('',#17782,#14309,#14310);
#13054=AXIS2_PLACEMENT_3D('',#17784,#14311,#14312);
#13055=AXIS2_PLACEMENT_3D('',#17787,#14314,#14315);
#13056=AXIS2_PLACEMENT_3D('',#17788,#14316,#14317);
#13057=AXIS2_PLACEMENT_3D('',#17789,#14318,#14319);
#13058=AXIS2_PLACEMENT_3D('',#17791,#14320,#14321);
#13059=AXIS2_PLACEMENT_3D('',#17794,#14323,#14324);
#13060=AXIS2_PLACEMENT_3D('',#17795,#14325,#14326);
#13061=AXIS2_PLACEMENT_3D('',#17796,#14327,#14328);
#13062=AXIS2_PLACEMENT_3D('',#17805,#14333,#14334);
#13063=AXIS2_PLACEMENT_3D('',#17814,#14339,#14340);
#13064=AXIS2_PLACEMENT_3D('',#17816,#14341,#14342);
#13065=AXIS2_PLACEMENT_3D('',#17823,#14346,#14347);
#13066=AXIS2_PLACEMENT_3D('',#17824,#14348,#14349);
#13067=AXIS2_PLACEMENT_3D('',#17825,#14350,#14351);
#13068=AXIS2_PLACEMENT_3D('',#17826,#14352,#14353);
#13069=AXIS2_PLACEMENT_3D('',#17827,#14354,#14355);
#13070=AXIS2_PLACEMENT_3D('',#17830,#14357,#14358);
#13071=AXIS2_PLACEMENT_3D('',#17831,#14359,#14360);
#13072=AXIS2_PLACEMENT_3D('',#17833,#14361,#14362);
#13073=AXIS2_PLACEMENT_3D('',#17835,#14364,#14365);
#13074=AXIS2_PLACEMENT_3D('',#17841,#14369,#14370);
#13075=AXIS2_PLACEMENT_3D('',#17843,#14372,#14373);
#13076=AXIS2_PLACEMENT_3D('',#17845,#14375,#14376);
#13077=AXIS2_PLACEMENT_3D('',#17847,#14377,#14378);
#13078=AXIS2_PLACEMENT_3D('',#17850,#14380,#14381);
#13079=AXIS2_PLACEMENT_3D('',#17851,#14382,#14383);
#13080=AXIS2_PLACEMENT_3D('',#17852,#14384,#14385);
#13081=AXIS2_PLACEMENT_3D('',#17854,#14386,#14387);
#13082=AXIS2_PLACEMENT_3D('',#17857,#14389,#14390);
#13083=AXIS2_PLACEMENT_3D('',#17858,#14391,#14392);
#13084=AXIS2_PLACEMENT_3D('',#17859,#14393,#14394);
#13085=AXIS2_PLACEMENT_3D('',#17868,#14399,#14400);
#13086=AXIS2_PLACEMENT_3D('',#17877,#14405,#14406);
#13087=AXIS2_PLACEMENT_3D('',#17879,#14407,#14408);
#13088=AXIS2_PLACEMENT_3D('',#17886,#14412,#14413);
#13089=AXIS2_PLACEMENT_3D('',#17887,#14414,#14415);
#13090=AXIS2_PLACEMENT_3D('',#17888,#14416,#14417);
#13091=AXIS2_PLACEMENT_3D('',#17889,#14418,#14419);
#13092=AXIS2_PLACEMENT_3D('',#17890,#14420,#14421);
#13093=AXIS2_PLACEMENT_3D('',#17893,#14423,#14424);
#13094=AXIS2_PLACEMENT_3D('',#17894,#14425,#14426);
#13095=AXIS2_PLACEMENT_3D('',#17896,#14427,#14428);
#13096=AXIS2_PLACEMENT_3D('',#17898,#14430,#14431);
#13097=AXIS2_PLACEMENT_3D('',#17904,#14435,#14436);
#13098=AXIS2_PLACEMENT_3D('',#17906,#14438,#14439);
#13099=AXIS2_PLACEMENT_3D('',#17908,#14441,#14442);
#13100=AXIS2_PLACEMENT_3D('',#17910,#14443,#14444);
#13101=AXIS2_PLACEMENT_3D('',#17913,#14446,#14447);
#13102=AXIS2_PLACEMENT_3D('',#17914,#14448,#14449);
#13103=AXIS2_PLACEMENT_3D('',#17916,#14450,#14451);
#13104=AXIS2_PLACEMENT_3D('',#17919,#14453,#14454);
#13105=AXIS2_PLACEMENT_3D('',#17920,#14455,#14456);
#13106=AXIS2_PLACEMENT_3D('',#17922,#14457,#14458);
#13107=AXIS2_PLACEMENT_3D('',#17925,#14460,#14461);
#13108=AXIS2_PLACEMENT_3D('',#17926,#14462,#14463);
#13109=AXIS2_PLACEMENT_3D('',#17928,#14464,#14465);
#13110=AXIS2_PLACEMENT_3D('',#17931,#14467,#14468);
#13111=AXIS2_PLACEMENT_3D('',#17932,#14469,#14470);
#13112=AXIS2_PLACEMENT_3D('',#17949,#14479,#14480);
#13113=AXIS2_PLACEMENT_3D('',#17955,#14484,#14485);
#13114=AXIS2_PLACEMENT_3D('',#17959,#14488,#14489);
#13115=AXIS2_PLACEMENT_3D('',#17963,#14492,#14493);
#13116=AXIS2_PLACEMENT_3D('',#17965,#14495,#14496);
#13117=AXIS2_PLACEMENT_3D('',#17971,#14500,#14501);
#13118=AXIS2_PLACEMENT_3D('',#17975,#14504,#14505);
#13119=AXIS2_PLACEMENT_3D('',#17979,#14508,#14509);
#13120=AXIS2_PLACEMENT_3D('',#17981,#14511,#14512);
#13121=AXIS2_PLACEMENT_3D('',#17982,#14513,#14514);
#14307=DIRECTION('axis',(0.,0.,1.));
#14308=DIRECTION('refdir',(1.,0.,0.));
#14309=DIRECTION('center_axis',(0.,0.,1.));
#14310=DIRECTION('ref_axis',(1.,0.,0.));
#14311=DIRECTION('center_axis',(0.,0.,1.));
#14312=DIRECTION('ref_axis',(1.,0.,0.));
#14313=DIRECTION('',(0.,0.,1.));
#14314=DIRECTION('center_axis',(0.,0.,-1.));
#14315=DIRECTION('ref_axis',(1.,0.,0.));
#14316=DIRECTION('center_axis',(0.,0.,1.));
#14317=DIRECTION('ref_axis',(1.,0.,0.));
#14318=DIRECTION('center_axis',(0.,0.,1.));
#14319=DIRECTION('ref_axis',(1.,0.,0.));
#14320=DIRECTION('center_axis',(0.,0.,1.));
#14321=DIRECTION('ref_axis',(1.,0.,0.));
#14322=DIRECTION('',(0.,0.,1.));
#14323=DIRECTION('center_axis',(0.,0.,-1.));
#14324=DIRECTION('ref_axis',(1.,0.,0.));
#14325=DIRECTION('center_axis',(0.,0.,1.));
#14326=DIRECTION('ref_axis',(1.,0.,0.));
#14327=DIRECTION('center_axis',(0.,1.,0.));
#14328=DIRECTION('ref_axis',(-1.,0.,0.));
#14329=DIRECTION('',(0.,0.,1.));
#14330=DIRECTION('',(-1.,0.,0.));
#14331=DIRECTION('',(0.,0.,-1.));
#14332=DIRECTION('',(1.,0.,0.));
#14333=DIRECTION('center_axis',(0.,-1.,0.));
#14334=DIRECTION('ref_axis',(1.,0.,0.));
#14335=DIRECTION('',(0.,0.,-1.));
#14336=DIRECTION('',(-1.,0.,0.));
#14337=DIRECTION('',(0.,0.,1.));
#14338=DIRECTION('',(1.,0.,0.));
#14339=DIRECTION('center_axis',(0.,0.,1.));
#14340=DIRECTION('ref_axis',(1.,0.,0.));
#14341=DIRECTION('center_axis',(0.,0.,1.));
#14342=DIRECTION('ref_axis',(1.,0.,0.));
#14343=DIRECTION('',(-1.,0.,0.));
#14344=DIRECTION('',(0.,1.,0.));
#14345=DIRECTION('',(1.,0.,0.));
#14346=DIRECTION('center_axis',(0.,0.,1.));
#14347=DIRECTION('ref_axis',(1.,0.,0.));
#14348=DIRECTION('center_axis',(0.,0.,1.));
#14349=DIRECTION('ref_axis',(1.,0.,0.));
#14350=DIRECTION('center_axis',(0.,0.,1.));
#14351=DIRECTION('ref_axis',(1.,0.,0.));
#14352=DIRECTION('center_axis',(0.,0.,-1.));
#14353=DIRECTION('ref_axis',(1.,0.,0.));
#14354=DIRECTION('center_axis',(0.,0.,1.));
#14355=DIRECTION('ref_axis',(1.,0.,0.));
#14356=DIRECTION('',(0.,0.,1.));
#14357=DIRECTION('center_axis',(0.,0.,1.));
#14358=DIRECTION('ref_axis',(1.,0.,0.));
#14359=DIRECTION('center_axis',(0.,0.,1.));
#14360=DIRECTION('ref_axis',(1.,0.,0.));
#14361=DIRECTION('center_axis',(0.,0.,1.));
#14362=DIRECTION('ref_axis',(1.,0.,0.));
#14363=DIRECTION('',(0.,0.,1.));
#14364=DIRECTION('center_axis',(0.,0.,1.));
#14365=DIRECTION('ref_axis',(1.,0.,0.));
#14366=DIRECTION('',(1.,0.,0.));
#14367=DIRECTION('',(0.,-1.,0.));
#14368=DIRECTION('',(-1.,0.,0.));
#14369=DIRECTION('center_axis',(0.,-1.,0.));
#14370=DIRECTION('ref_axis',(1.,0.,0.));
#14371=DIRECTION('',(0.,0.,-1.));
#14372=DIRECTION('center_axis',(0.,1.,0.));
#14373=DIRECTION('ref_axis',(-1.,0.,0.));
#14374=DIRECTION('',(0.,0.,1.));
#14375=DIRECTION('center_axis',(0.,0.,1.));
#14376=DIRECTION('ref_axis',(1.,0.,0.));
#14377=DIRECTION('center_axis',(0.,0.,1.));
#14378=DIRECTION('ref_axis',(1.,0.,0.));
#14379=DIRECTION('',(0.,0.,1.));
#14380=DIRECTION('center_axis',(0.,0.,-1.));
#14381=DIRECTION('ref_axis',(1.,0.,0.));
#14382=DIRECTION('center_axis',(0.,0.,1.));
#14383=DIRECTION('ref_axis',(1.,0.,0.));
#14384=DIRECTION('center_axis',(0.,0.,1.));
#14385=DIRECTION('ref_axis',(1.,0.,0.));
#14386=DIRECTION('center_axis',(0.,0.,1.));
#14387=DIRECTION('ref_axis',(1.,0.,0.));
#14388=DIRECTION('',(0.,0.,1.));
#14389=DIRECTION('center_axis',(0.,0.,-1.));
#14390=DIRECTION('ref_axis',(1.,0.,0.));
#14391=DIRECTION('center_axis',(0.,0.,1.));
#14392=DIRECTION('ref_axis',(1.,0.,0.));
#14393=DIRECTION('center_axis',(0.,1.,0.));
#14394=DIRECTION('ref_axis',(-1.,0.,0.));
#14395=DIRECTION('',(0.,0.,1.));
#14396=DIRECTION('',(-1.,0.,0.));
#14397=DIRECTION('',(0.,0.,-1.));
#14398=DIRECTION('',(1.,0.,0.));
#14399=DIRECTION('center_axis',(0.,-1.,0.));
#14400=DIRECTION('ref_axis',(1.,0.,0.));
#14401=DIRECTION('',(0.,0.,-1.));
#14402=DIRECTION('',(-1.,0.,0.));
#14403=DIRECTION('',(0.,0.,1.));
#14404=DIRECTION('',(1.,0.,0.));
#14405=DIRECTION('center_axis',(0.,0.,1.));
#14406=DIRECTION('ref_axis',(1.,0.,0.));
#14407=DIRECTION('center_axis',(0.,0.,1.));
#14408=DIRECTION('ref_axis',(1.,0.,0.));
#14409=DIRECTION('',(-1.,0.,0.));
#14410=DIRECTION('',(0.,1.,0.));
#14411=DIRECTION('',(1.,0.,0.));
#14412=DIRECTION('center_axis',(0.,0.,1.));
#14413=DIRECTION('ref_axis',(1.,0.,0.));
#14414=DIRECTION('center_axis',(0.,0.,1.));
#14415=DIRECTION('ref_axis',(1.,0.,0.));
#14416=DIRECTION('center_axis',(0.,0.,1.));
#14417=DIRECTION('ref_axis',(1.,0.,0.));
#14418=DIRECTION('center_axis',(0.,0.,-1.));
#14419=DIRECTION('ref_axis',(1.,0.,0.));
#14420=DIRECTION('center_axis',(0.,0.,1.));
#14421=DIRECTION('ref_axis',(1.,0.,0.));
#14422=DIRECTION('',(0.,0.,1.));
#14423=DIRECTION('center_axis',(0.,0.,1.));
#14424=DIRECTION('ref_axis',(1.,0.,0.));
#14425=DIRECTION('center_axis',(0.,0.,1.));
#14426=DIRECTION('ref_axis',(1.,0.,0.));
#14427=DIRECTION('center_axis',(0.,0.,1.));
#14428=DIRECTION('ref_axis',(1.,0.,0.));
#14429=DIRECTION('',(0.,0.,1.));
#14430=DIRECTION('center_axis',(0.,0.,1.));
#14431=DIRECTION('ref_axis',(1.,0.,0.));
#14432=DIRECTION('',(1.,0.,0.));
#14433=DIRECTION('',(0.,-1.,0.));
#14434=DIRECTION('',(-1.,0.,0.));
#14435=DIRECTION('center_axis',(0.,-1.,0.));
#14436=DIRECTION('ref_axis',(1.,0.,0.));
#14437=DIRECTION('',(0.,0.,-1.));
#14438=DIRECTION('center_axis',(0.,1.,0.));
#14439=DIRECTION('ref_axis',(-1.,0.,0.));
#14440=DIRECTION('',(0.,0.,1.));
#14441=DIRECTION('center_axis',(0.,0.,1.));
#14442=DIRECTION('ref_axis',(1.,0.,0.));
#14443=DIRECTION('center_axis',(0.,0.,1.));
#14444=DIRECTION('ref_axis',(1.,0.,0.));
#14445=DIRECTION('',(0.,0.,1.));
#14446=DIRECTION('center_axis',(0.,0.,-1.));
#14447=DIRECTION('ref_axis',(1.,0.,0.));
#14448=DIRECTION('center_axis',(0.,0.,1.));
#14449=DIRECTION('ref_axis',(1.,0.,0.));
#14450=DIRECTION('center_axis',(0.,0.,1.));
#14451=DIRECTION('ref_axis',(1.,0.,0.));
#14452=DIRECTION('',(0.,0.,1.));
#14453=DIRECTION('center_axis',(0.,0.,-1.));
#14454=DIRECTION('ref_axis',(1.,0.,0.));
#14455=DIRECTION('center_axis',(0.,0.,1.));
#14456=DIRECTION('ref_axis',(1.,0.,0.));
#14457=DIRECTION('center_axis',(0.,0.,1.));
#14458=DIRECTION('ref_axis',(1.,0.,0.));
#14459=DIRECTION('',(0.,0.,1.));
#14460=DIRECTION('center_axis',(0.,0.,-1.));
#14461=DIRECTION('ref_axis',(1.,0.,0.));
#14462=DIRECTION('center_axis',(0.,0.,1.));
#14463=DIRECTION('ref_axis',(1.,0.,0.));
#14464=DIRECTION('center_axis',(0.,0.,1.));
#14465=DIRECTION('ref_axis',(1.,0.,0.));
#14466=DIRECTION('',(0.,0.,1.));
#14467=DIRECTION('center_axis',(0.,0.,-1.));
#14468=DIRECTION('ref_axis',(1.,0.,0.));
#14469=DIRECTION('center_axis',(0.,0.,1.));
#14470=DIRECTION('ref_axis',(1.,0.,0.));
#14471=DIRECTION('',(0.,-1.,0.));
#14472=DIRECTION('',(1.,0.,0.));
#14473=DIRECTION('',(0.,1.,0.));
#14474=DIRECTION('',(-1.,0.,0.));
#14475=DIRECTION('',(-1.,0.,0.));
#14476=DIRECTION('',(0.,1.,0.));
#14477=DIRECTION('',(1.,0.,0.));
#14478=DIRECTION('',(0.,-1.,0.));
#14479=DIRECTION('center_axis',(0.,1.,0.));
#14480=DIRECTION('ref_axis',(-1.,0.,0.));
#14481=DIRECTION('',(-1.,0.,0.));
#14482=DIRECTION('',(0.,0.,1.));
#14483=DIRECTION('',(0.,0.,1.));
#14484=DIRECTION('center_axis',(1.,0.,0.));
#14485=DIRECTION('ref_axis',(0.,1.,0.));
#14486=DIRECTION('',(0.,1.,0.));
#14487=DIRECTION('',(0.,0.,1.));
#14488=DIRECTION('center_axis',(0.,-1.,0.));
#14489=DIRECTION('ref_axis',(1.,0.,0.));
#14490=DIRECTION('',(1.,0.,0.));
#14491=DIRECTION('',(0.,0.,1.));
#14492=DIRECTION('center_axis',(-1.,0.,0.));
#14493=DIRECTION('ref_axis',(0.,-1.,0.));
#14494=DIRECTION('',(0.,-1.,0.));
#14495=DIRECTION('center_axis',(0.,-1.,0.));
#14496=DIRECTION('ref_axis',(1.,0.,0.));
#14497=DIRECTION('',(0.,0.,1.));
#14498=DIRECTION('',(1.,0.,0.));
#14499=DIRECTION('',(0.,0.,1.));
#14500=DIRECTION('center_axis',(1.,0.,0.));
#14501=DIRECTION('ref_axis',(0.,1.,0.));
#14502=DIRECTION('',(0.,0.,1.));
#14503=DIRECTION('',(0.,1.,0.));
#14504=DIRECTION('center_axis',(0.,1.,0.));
#14505=DIRECTION('ref_axis',(-1.,0.,0.));
#14506=DIRECTION('',(0.,0.,1.));
#14507=DIRECTION('',(-1.,0.,0.));
#14508=DIRECTION('center_axis',(-1.,0.,0.));
#14509=DIRECTION('ref_axis',(0.,-1.,0.));
#14510=DIRECTION('',(0.,-1.,0.));
#14511=DIRECTION('center_axis',(0.,0.,1.));
#14512=DIRECTION('ref_axis',(1.,0.,0.));
#14513=DIRECTION('center_axis',(0.,0.,1.));
#14514=DIRECTION('ref_axis',(1.,0.,0.));
#17781=CARTESIAN_POINT('',(0.,0.,0.));
#17782=CARTESIAN_POINT('Origin',(2.4,-1.6,24.4));
#17783=CARTESIAN_POINT('',(2.235,-1.6,24.4));
#17784=CARTESIAN_POINT('Origin',(2.4,-1.6,24.4));
#17785=CARTESIAN_POINT('',(2.235,-1.6,25.));
#17786=CARTESIAN_POINT('',(2.235,-1.6,24.4));
#17787=CARTESIAN_POINT('Origin',(2.4,-1.6,25.));
#17788=CARTESIAN_POINT('Origin',(2.4,-1.6,24.4));
#17789=CARTESIAN_POINT('Origin',(2.4,1.6,24.4));
#17790=CARTESIAN_POINT('',(2.235,1.6,24.4));
#17791=CARTESIAN_POINT('Origin',(2.4,1.6,24.4));
#17792=CARTESIAN_POINT('',(2.235,1.6,25.));
#17793=CARTESIAN_POINT('',(2.235,1.6,24.4));
#17794=CARTESIAN_POINT('Origin',(2.4,1.6,25.));
#17795=CARTESIAN_POINT('Origin',(2.4,1.6,24.4));
#17796=CARTESIAN_POINT('Origin',(0.21,1.01,22.9));
#17797=CARTESIAN_POINT('',(-0.726238685697896,1.01,23.));
#17798=CARTESIAN_POINT('',(-0.726238685697896,1.01,25.));
#17799=CARTESIAN_POINT('',(-0.726238685697896,1.01,23.));
#17800=CARTESIAN_POINT('',(0.0305156009506911,1.01,23.));
#17801=CARTESIAN_POINT('',(1.98,1.01,23.));
#17802=CARTESIAN_POINT('',(0.0305156009506911,1.01,25.));
#17803=CARTESIAN_POINT('',(0.0305156009506911,1.01,22.9));
#17804=CARTESIAN_POINT('',(1.98,1.01,25.));
#17805=CARTESIAN_POINT('Origin',(-1.1,-1.01,22.9));
#17806=CARTESIAN_POINT('',(-0.726238685697896,-1.01,25.));
#17807=CARTESIAN_POINT('',(-0.726238685697896,-1.01,23.));
#17808=CARTESIAN_POINT('',(-0.726238685697896,-1.01,23.));
#17809=CARTESIAN_POINT('',(0.0305156009506911,-1.01,25.));
#17810=CARTESIAN_POINT('',(1.325,-1.01,25.));
#17811=CARTESIAN_POINT('',(0.0305156009506911,-1.01,23.));
#17812=CARTESIAN_POINT('',(0.0305156009506911,-1.01,22.9));
#17813=CARTESIAN_POINT('',(1.325,-1.01,23.));
#17814=CARTESIAN_POINT('Origin',(3.75,0.,23.));
#17815=CARTESIAN_POINT('',(1.,2.,23.));
#17816=CARTESIAN_POINT('Origin',(1.,0.,23.));
#17817=CARTESIAN_POINT('',(4.5,2.,23.));
#17818=CARTESIAN_POINT('',(6.5,2.,23.));
#17819=CARTESIAN_POINT('',(4.5,-2.,23.));
#17820=CARTESIAN_POINT('',(4.5,1.25,23.));
#17821=CARTESIAN_POINT('',(1.,-2.,23.));
#17822=CARTESIAN_POINT('',(1.,-2.,23.));
#17823=CARTESIAN_POINT('Origin',(1.,0.,23.));
#17824=CARTESIAN_POINT('Origin',(1.,0.,23.));
#17825=CARTESIAN_POINT('Origin',(1.,0.,22.9));
#17826=CARTESIAN_POINT('Origin',(1.,0.,25.));
#17827=CARTESIAN_POINT('Origin',(1.,0.,23.));
#17828=CARTESIAN_POINT('',(1.,-2.,25.));
#17829=CARTESIAN_POINT('',(1.,-2.,23.));
#17830=CARTESIAN_POINT('Origin',(1.,0.,25.));
#17831=CARTESIAN_POINT('Origin',(1.,0.,23.));
#17832=CARTESIAN_POINT('',(1.,2.,25.));
#17833=CARTESIAN_POINT('Origin',(1.,0.,25.));
#17834=CARTESIAN_POINT('',(1.,2.,23.));
#17835=CARTESIAN_POINT('Origin',(3.75,0.,25.));
#17836=CARTESIAN_POINT('',(4.5,-2.,25.));
#17837=CARTESIAN_POINT('',(1.,-2.,25.));
#17838=CARTESIAN_POINT('',(4.5,2.,25.));
#17839=CARTESIAN_POINT('',(4.5,1.25,25.));
#17840=CARTESIAN_POINT('',(6.5,2.,25.));
#17841=CARTESIAN_POINT('Origin',(1.,-2.,23.));
#17842=CARTESIAN_POINT('',(4.5,-2.,12.));
#17843=CARTESIAN_POINT('Origin',(6.5,2.,23.));
#17844=CARTESIAN_POINT('',(4.5,2.,12.));
#17845=CARTESIAN_POINT('Origin',(2.4,-1.6,14.4));
#17846=CARTESIAN_POINT('',(2.235,-1.6,14.4));
#17847=CARTESIAN_POINT('Origin',(2.4,-1.6,14.4));
#17848=CARTESIAN_POINT('',(2.235,-1.6,15.));
#17849=CARTESIAN_POINT('',(2.235,-1.6,14.4));
#17850=CARTESIAN_POINT('Origin',(2.4,-1.6,15.));
#17851=CARTESIAN_POINT('Origin',(2.4,-1.6,14.4));
#17852=CARTESIAN_POINT('Origin',(2.4,1.6,14.4));
#17853=CARTESIAN_POINT('',(2.235,1.6,14.4));
#17854=CARTESIAN_POINT('Origin',(2.4,1.6,14.4));
#17855=CARTESIAN_POINT('',(2.235,1.6,15.));
#17856=CARTESIAN_POINT('',(2.235,1.6,14.4));
#17857=CARTESIAN_POINT('Origin',(2.4,1.6,15.));
#17858=CARTESIAN_POINT('Origin',(2.4,1.6,14.4));
#17859=CARTESIAN_POINT('Origin',(0.21,1.01,12.9));
#17860=CARTESIAN_POINT('',(-0.726238685697896,1.01,13.));
#17861=CARTESIAN_POINT('',(-0.726238685697896,1.01,15.));
#17862=CARTESIAN_POINT('',(-0.726238685697896,1.01,13.));
#17863=CARTESIAN_POINT('',(0.0305156009506911,1.01,13.));
#17864=CARTESIAN_POINT('',(1.98,1.01,13.));
#17865=CARTESIAN_POINT('',(0.0305156009506911,1.01,15.));
#17866=CARTESIAN_POINT('',(0.0305156009506911,1.01,12.9));
#17867=CARTESIAN_POINT('',(1.98,1.01,15.));
#17868=CARTESIAN_POINT('Origin',(-1.1,-1.01,12.9));
#17869=CARTESIAN_POINT('',(-0.726238685697896,-1.01,15.));
#17870=CARTESIAN_POINT('',(-0.726238685697896,-1.01,13.));
#17871=CARTESIAN_POINT('',(-0.726238685697896,-1.01,13.));
#17872=CARTESIAN_POINT('',(0.0305156009506911,-1.01,15.));
#17873=CARTESIAN_POINT('',(1.325,-1.01,15.));
#17874=CARTESIAN_POINT('',(0.0305156009506911,-1.01,13.));
#17875=CARTESIAN_POINT('',(0.0305156009506911,-1.01,12.9));
#17876=CARTESIAN_POINT('',(1.325,-1.01,13.));
#17877=CARTESIAN_POINT('Origin',(3.75,0.,13.));
#17878=CARTESIAN_POINT('',(1.,2.,13.));
#17879=CARTESIAN_POINT('Origin',(1.,0.,13.));
#17880=CARTESIAN_POINT('',(4.5,2.,13.));
#17881=CARTESIAN_POINT('',(6.5,2.,13.));
#17882=CARTESIAN_POINT('',(4.5,-2.,13.));
#17883=CARTESIAN_POINT('',(4.5,1.25,13.));
#17884=CARTESIAN_POINT('',(1.,-2.,13.));
#17885=CARTESIAN_POINT('',(1.,-2.,13.));
#17886=CARTESIAN_POINT('Origin',(1.,0.,13.));
#17887=CARTESIAN_POINT('Origin',(1.,0.,13.));
#17888=CARTESIAN_POINT('Origin',(1.,0.,12.9));
#17889=CARTESIAN_POINT('Origin',(1.,0.,15.));
#17890=CARTESIAN_POINT('Origin',(1.,0.,13.));
#17891=CARTESIAN_POINT('',(1.,-2.,15.));
#17892=CARTESIAN_POINT('',(1.,-2.,13.));
#17893=CARTESIAN_POINT('Origin',(1.,0.,15.));
#17894=CARTESIAN_POINT('Origin',(1.,0.,13.));
#17895=CARTESIAN_POINT('',(1.,2.,15.));
#17896=CARTESIAN_POINT('Origin',(1.,0.,15.));
#17897=CARTESIAN_POINT('',(1.,2.,13.));
#17898=CARTESIAN_POINT('Origin',(3.75,0.,15.));
#17899=CARTESIAN_POINT('',(4.5,-2.,15.));
#17900=CARTESIAN_POINT('',(1.,-2.,15.));
#17901=CARTESIAN_POINT('',(4.5,2.,15.));
#17902=CARTESIAN_POINT('',(4.5,1.25,15.));
#17903=CARTESIAN_POINT('',(6.5,2.,15.));
#17904=CARTESIAN_POINT('Origin',(1.,-2.,13.));
#17905=CARTESIAN_POINT('',(4.5,-2.,7.));
#17906=CARTESIAN_POINT('Origin',(6.5,2.,13.));
#17907=CARTESIAN_POINT('',(4.5,2.,7.));
#17908=CARTESIAN_POINT('Origin',(7.,-3.2,0.9));
#17909=CARTESIAN_POINT('',(6.725,-3.2,1.));
#17910=CARTESIAN_POINT('Origin',(7.,-3.2,1.));
#17911=CARTESIAN_POINT('',(6.725,-3.2,2.));
#17912=CARTESIAN_POINT('',(6.725,-3.2,0.9));
#17913=CARTESIAN_POINT('Origin',(7.,-3.2,2.));
#17914=CARTESIAN_POINT('Origin',(4.,3.2,0.9));
#17915=CARTESIAN_POINT('',(3.725,3.2,1.));
#17916=CARTESIAN_POINT('Origin',(4.,3.2,1.));
#17917=CARTESIAN_POINT('',(3.725,3.2,2.));
#17918=CARTESIAN_POINT('',(3.725,3.2,0.9));
#17919=CARTESIAN_POINT('Origin',(4.,3.2,2.));
#17920=CARTESIAN_POINT('Origin',(4.,-3.2,0.9));
#17921=CARTESIAN_POINT('',(3.725,-3.2,1.));
#17922=CARTESIAN_POINT('Origin',(4.,-3.2,1.));
#17923=CARTESIAN_POINT('',(3.725,-3.2,2.));
#17924=CARTESIAN_POINT('',(3.725,-3.2,0.9));
#17925=CARTESIAN_POINT('Origin',(4.,-3.2,2.));
#17926=CARTESIAN_POINT('Origin',(7.,3.2,0.9));
#17927=CARTESIAN_POINT('',(6.725,3.2,1.));
#17928=CARTESIAN_POINT('Origin',(7.,3.2,1.));
#17929=CARTESIAN_POINT('',(6.725,3.2,2.));
#17930=CARTESIAN_POINT('',(6.725,3.2,0.9));
#17931=CARTESIAN_POINT('Origin',(7.,3.2,2.));
#17932=CARTESIAN_POINT('Origin',(5.5,0.,2.));
#17933=CARTESIAN_POINT('',(3.5,4.,2.));
#17934=CARTESIAN_POINT('',(3.5,-4.,2.));
#17935=CARTESIAN_POINT('',(3.5,4.,2.));
#17936=CARTESIAN_POINT('',(7.5,-4.,2.));
#17937=CARTESIAN_POINT('',(3.5,-4.,2.));
#17938=CARTESIAN_POINT('',(7.5,4.,2.));
#17939=CARTESIAN_POINT('',(7.5,-4.,2.));
#17940=CARTESIAN_POINT('',(7.5,4.,2.));
#17941=CARTESIAN_POINT('',(6.5,2.5,2.));
#17942=CARTESIAN_POINT('',(4.5,2.5,2.));
#17943=CARTESIAN_POINT('',(6.,2.5,2.));
#17944=CARTESIAN_POINT('',(6.5,-2.5,2.));
#17945=CARTESIAN_POINT('',(6.5,-1.25,2.));
#17946=CARTESIAN_POINT('',(4.5,-2.5,2.));
#17947=CARTESIAN_POINT('',(5.,-2.5,2.));
#17948=CARTESIAN_POINT('',(4.5,1.25,2.));
#17949=CARTESIAN_POINT('Origin',(7.5,4.,1.));
#17950=CARTESIAN_POINT('',(7.5,4.,1.));
#17951=CARTESIAN_POINT('',(3.5,4.,1.));
#17952=CARTESIAN_POINT('',(7.5,4.,1.));
#17953=CARTESIAN_POINT('',(3.5,4.,1.));
#17954=CARTESIAN_POINT('',(7.5,4.,1.));
#17955=CARTESIAN_POINT('Origin',(7.5,-4.,1.));
#17956=CARTESIAN_POINT('',(7.5,-4.,1.));
#17957=CARTESIAN_POINT('',(7.5,-4.,1.));
#17958=CARTESIAN_POINT('',(7.5,-4.,1.));
#17959=CARTESIAN_POINT('Origin',(3.5,-4.,1.));
#17960=CARTESIAN_POINT('',(3.5,-4.,1.));
#17961=CARTESIAN_POINT('',(3.5,-4.,1.));
#17962=CARTESIAN_POINT('',(3.5,-4.,1.));
#17963=CARTESIAN_POINT('Origin',(3.5,4.,1.));
#17964=CARTESIAN_POINT('',(3.5,4.,1.));
#17965=CARTESIAN_POINT('Origin',(4.5,-2.5,1.));
#17966=CARTESIAN_POINT('',(6.5,-2.5,31.));
#17967=CARTESIAN_POINT('',(6.5,-2.5,1.));
#17968=CARTESIAN_POINT('',(4.5,-2.5,31.));
#17969=CARTESIAN_POINT('',(4.5,-2.5,31.));
#17970=CARTESIAN_POINT('',(4.5,-2.5,1.));
#17971=CARTESIAN_POINT('Origin',(6.5,-2.5,1.));
#17972=CARTESIAN_POINT('',(6.5,2.5,31.));
#17973=CARTESIAN_POINT('',(6.5,2.5,1.));
#17974=CARTESIAN_POINT('',(6.5,-2.5,31.));
#17975=CARTESIAN_POINT('Origin',(6.5,2.5,1.));
#17976=CARTESIAN_POINT('',(4.5,2.5,31.));
#17977=CARTESIAN_POINT('',(4.5,2.5,1.));
#17978=CARTESIAN_POINT('',(6.5,2.5,31.));
#17979=CARTESIAN_POINT('Origin',(4.5,2.5,1.));
#17980=CARTESIAN_POINT('',(4.5,2.5,31.));
#17981=CARTESIAN_POINT('Origin',(5.5,0.,31.));
#17982=CARTESIAN_POINT('Origin',(5.5,0.,1.));
#32659=UNCERTAINTY_MEASURE_WITH_UNIT(LENGTH_MEASURE(0.001),#32752,
'DISTANCE_ACCURACY_VALUE',
'Maximum model space distance between geometric entities at asserted c
onnectivities');
#32702=UNCERTAINTY_MEASURE_WITH_UNIT(LENGTH_MEASURE(0.001),#32752,
'DISTANCE_ACCURACY_VALUE',
'Maximum model space distance between geometric entities at asserted c
onnectivities');
#32708=(
GEOMETRIC_REPRESENTATION_CONTEXT(3)
GLOBAL_UNCERTAINTY_ASSIGNED_CONTEXT((#32659))
GLOBAL_UNIT_ASSIGNED_CONTEXT((#32752,#32754,#32755))
REPRESENTATION_CONTEXT('','3D')
);
#32751=(
GEOMETRIC_REPRESENTATION_CONTEXT(3)
GLOBAL_UNCERTAINTY_ASSIGNED_CONTEXT((#32702))
GLOBAL_UNIT_ASSIGNED_CONTEXT((#32752,#32754,#32755))
REPRESENTATION_CONTEXT('','3D')
);
#32752=(
LENGTH_UNIT()
NAMED_UNIT(*)
SI_UNIT(.CENTI.,.METRE.)
);
#32754=(
NAMED_UNIT(*)
PLANE_ANGLE_UNIT()
SI_UNIT($,.RADIAN.)
);
#32755=(
NAMED_UNIT(*)
SI_UNIT($,.STERADIAN.)
SOLID_ANGLE_UNIT()
);
#32761=SHAPE_DEFINITION_REPRESENTATION(#32809,#32934);
#32809=PRODUCT_DEFINITION_SHAPE('',$,#32983);
#32934=SHAPE_REPRESENTATION('',(#13052),#32708);
#32977=PRODUCT_DEFINITION_CONTEXT('part definition',#33123,'design');
#32983=PRODUCT_DEFINITION('C frame','C frame',#33031,#32977);
#33031=PRODUCT_DEFINITION_FORMATION('',$,#33130);
#33123=APPLICATION_CONTEXT(
'Core Data for Automotive Mechanical Design Process');
#33124=PRODUCT_CONTEXT('part definition',#33123,'mechanical');
#33130=PRODUCT('C frame','C frame','C frame',(#33124));
#33215=COLOUR_RGB('Dark Blue',0.08,0.2,0.34);
#33216=FILL_AREA_STYLE_COLOUR('',#33215);
#33217=FILL_AREA_STYLE('',(#33216));
#33218=SURFACE_STYLE_FILL_AREA(#33217);
#33219=SURFACE_SIDE_STYLE('',(#33218));
#33220=SURFACE_STYLE_USAGE(.BOTH.,#33219);
#33221=PRESENTATION_STYLE_ASSIGNMENT((#33220));
ENDSEC;
END-ISO-10303-21;
